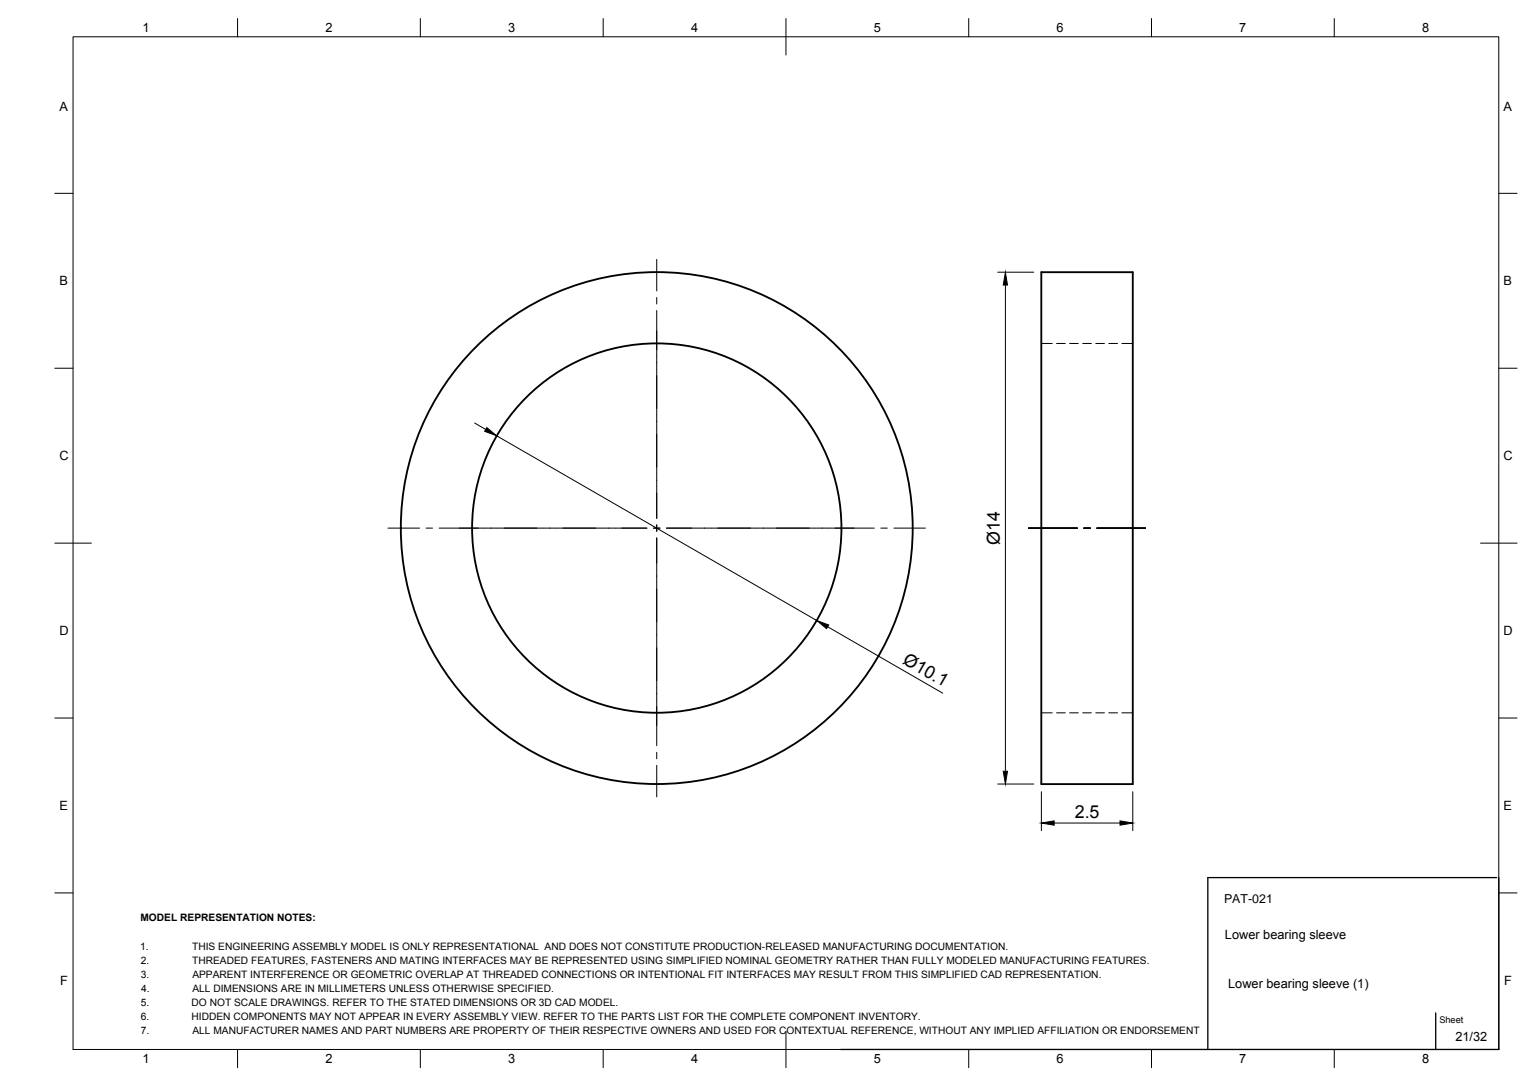
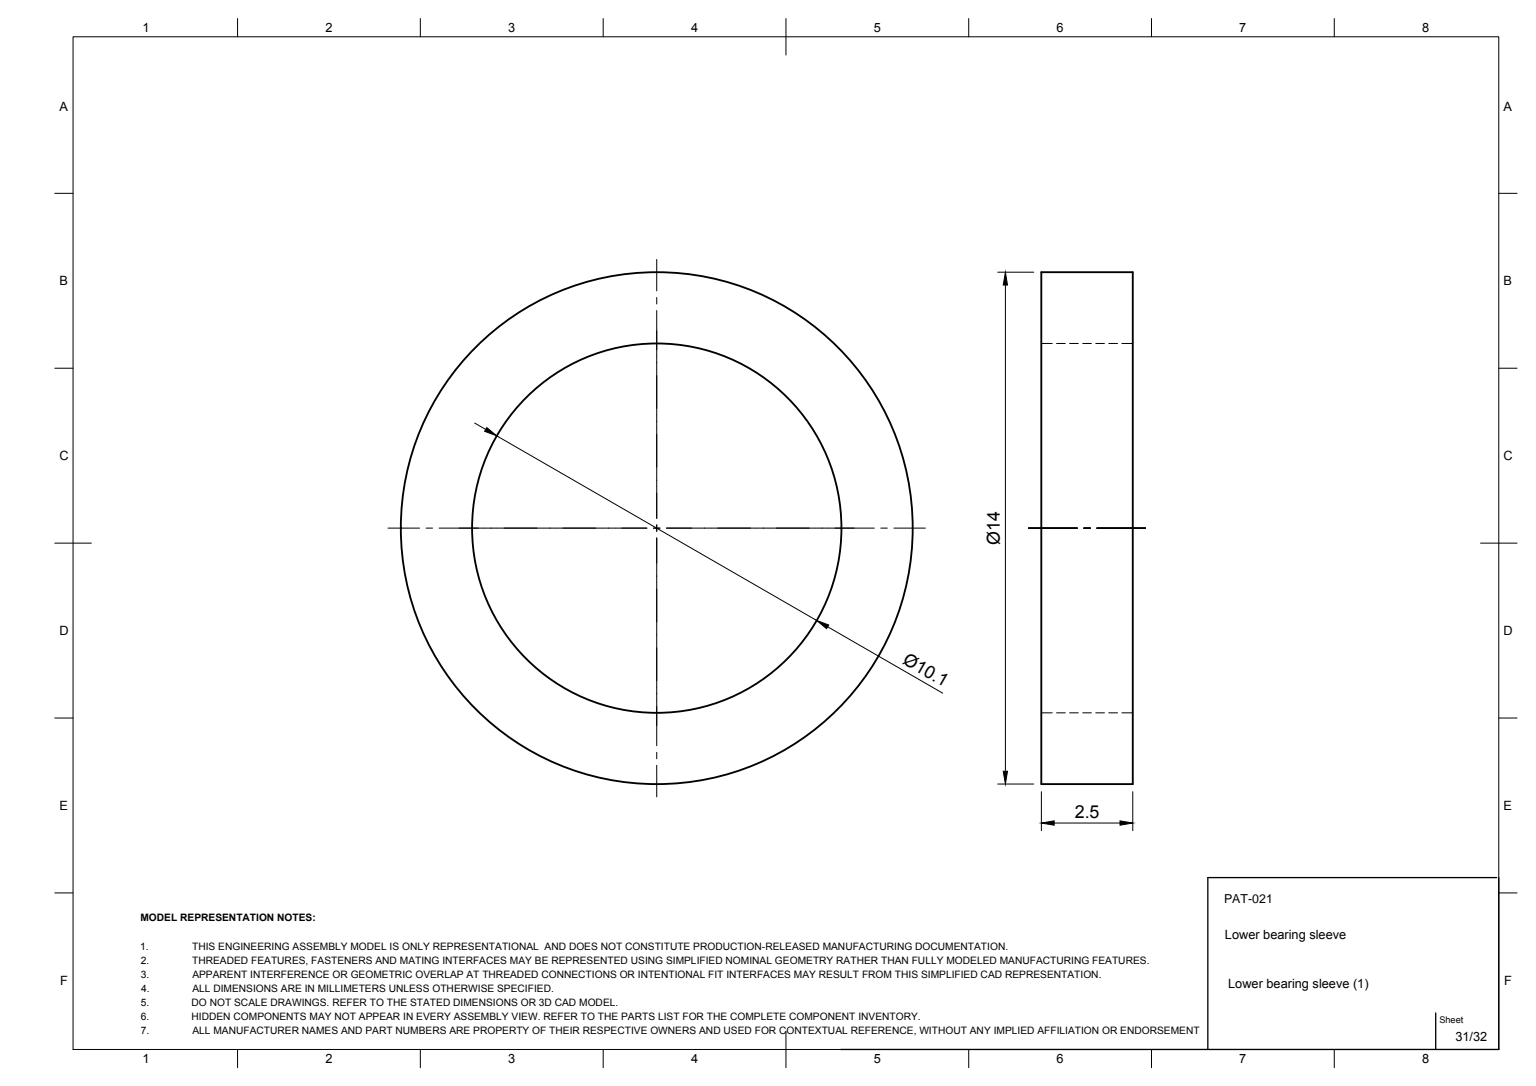
ISO-10303-21;
HEADER;
/* Generated by software containing ST-Developer
 * from STEP Tools, Inc. (www.steptools.com) 
 */

FILE_DESCRIPTION(
/* description */ ('Chain-less indexing wheel (Geneva) drive'),
/* implementation_level */ '2;1');

FILE_NAME(
/* name */ 'Lower bearing sleeve.step',
/* time_stamp */ '2026-10-28T03:25:22-07:00',
/* author */ (''),
/* organization */ (''),
/* preprocessor_version */ 'ST-DEVELOPER v20.2',
/* originating_system */ 'Autodesk Translation Framework v15.17.0.0',
/* authorisation */ '');

FILE_SCHEMA (('AUTOMOTIVE_DESIGN { 1 0 10303 214 3 1 1 }'));
ENDSEC;

DATA;
#10=MECHANICAL_DESIGN_GEOMETRIC_PRESENTATION_REPRESENTATION('',(#324),#10957);
#266=SHAPE_REPRESENTATION_RELATIONSHIP('SRR','None',#11081,#291);
#291=ADVANCED_BREP_SHAPE_REPRESENTATION('',(#356),#10944);
#324=STYLED_ITEM('',(#11287),#356);
#356=MANIFOLD_SOLID_BREP('Body1',#5721);
#439=FACE_BOUND('',#1255,.T.);
#440=FACE_BOUND('',#1257,.T.);
#567=PLANE('',#6448);
#568=PLANE('',#6449);
#847=FACE_OUTER_BOUND('',#1252,.T.);
#848=FACE_OUTER_BOUND('',#1253,.T.);
#849=FACE_OUTER_BOUND('',#1254,.T.);
#850=FACE_OUTER_BOUND('',#1256,.T.);
#1252=EDGE_LOOP('',(#4589,#4590,#4591,#4592));
#1253=EDGE_LOOP('',(#4593,#4594,#4595,#4596));
#1254=EDGE_LOOP('',(#4597));
#1255=EDGE_LOOP('',(#4598));
#1256=EDGE_LOOP('',(#4599));
#1257=EDGE_LOOP('',(#4600));
#1610=LINE('',#9926,#1984);
#1611=LINE('',#9932,#1985);
#1984=VECTOR('',#7804,0.505);
#1985=VECTOR('',#7811,0.7);
#2385=CIRCLE('',#6443,0.505);
#2386=CIRCLE('',#6444,0.505);
#2387=CIRCLE('',#6446,0.7);
#2388=CIRCLE('',#6447,0.7);
#2783=VERTEX_POINT('',#9923);
#2784=VERTEX_POINT('',#9925);
#2785=VERTEX_POINT('',#9929);
#2786=VERTEX_POINT('',#9931);
#3420=EDGE_CURVE('',#2783,#2783,#2385,.T.);
#3421=EDGE_CURVE('',#2783,#2784,#1610,.T.);
#3422=EDGE_CURVE('',#2784,#2784,#2386,.T.);
#3423=EDGE_CURVE('',#2785,#2785,#2387,.T.);
#3424=EDGE_CURVE('',#2785,#2786,#1611,.T.);
#3425=EDGE_CURVE('',#2786,#2786,#2388,.T.);
#4589=ORIENTED_EDGE('',*,*,#3420,.F.);
#4590=ORIENTED_EDGE('',*,*,#3421,.T.);
#4591=ORIENTED_EDGE('',*,*,#3422,.T.);
#4592=ORIENTED_EDGE('',*,*,#3421,.F.);
#4593=ORIENTED_EDGE('',*,*,#3423,.F.);
#4594=ORIENTED_EDGE('',*,*,#3424,.T.);
#4595=ORIENTED_EDGE('',*,*,#3425,.T.);
#4596=ORIENTED_EDGE('',*,*,#3424,.F.);
#4597=ORIENTED_EDGE('',*,*,#3423,.T.);
#4598=ORIENTED_EDGE('',*,*,#3420,.T.);
#4599=ORIENTED_EDGE('',*,*,#3425,.F.);
#4600=ORIENTED_EDGE('',*,*,#3422,.F.);
#5317=CYLINDRICAL_SURFACE('',#6442,0.505);
#5318=CYLINDRICAL_SURFACE('',#6445,0.7);
#5561=ADVANCED_FACE('',(#847),#5317,.F.);
#5562=ADVANCED_FACE('',(#848),#5318,.T.);
#5563=ADVANCED_FACE('',(#849,#439),#567,.T.);
#5564=ADVANCED_FACE('',(#850,#440),#568,.F.);
#5721=CLOSED_SHELL('',(#5561,#5562,#5563,#5564));
#6441=AXIS2_PLACEMENT_3D('',#9921,#7798,#7799);
#6442=AXIS2_PLACEMENT_3D('',#9922,#7800,#7801);
#6443=AXIS2_PLACEMENT_3D('',#9924,#7802,#7803);
#6444=AXIS2_PLACEMENT_3D('',#9927,#7805,#7806);
#6445=AXIS2_PLACEMENT_3D('',#9928,#7807,#7808);
#6446=AXIS2_PLACEMENT_3D('',#9930,#7809,#7810);
#6447=AXIS2_PLACEMENT_3D('',#9933,#7812,#7813);
#6448=AXIS2_PLACEMENT_3D('',#9934,#7814,#7815);
#6449=AXIS2_PLACEMENT_3D('',#9935,#7816,#7817);
#7798=DIRECTION('axis',(0.,0.,1.));
#7799=DIRECTION('refdir',(1.,0.,0.));
#7800=DIRECTION('center_axis',(0.,0.,1.));
#7801=DIRECTION('ref_axis',(1.,0.,0.));
#7802=DIRECTION('center_axis',(0.,0.,-1.));
#7803=DIRECTION('ref_axis',(1.,0.,0.));
#7804=DIRECTION('',(0.,0.,-1.));
#7805=DIRECTION('center_axis',(0.,0.,-1.));
#7806=DIRECTION('ref_axis',(1.,0.,0.));
#7807=DIRECTION('center_axis',(0.,0.,1.));
#7808=DIRECTION('ref_axis',(1.,0.,0.));
#7809=DIRECTION('center_axis',(0.,0.,1.));
#7810=DIRECTION('ref_axis',(1.,0.,0.));
#7811=DIRECTION('',(0.,0.,-1.));
#7812=DIRECTION('center_axis',(0.,0.,1.));
#7813=DIRECTION('ref_axis',(1.,0.,0.));
#7814=DIRECTION('center_axis',(0.,0.,1.));
#7815=DIRECTION('ref_axis',(1.,0.,0.));
#7816=DIRECTION('center_axis',(0.,0.,1.));
#7817=DIRECTION('ref_axis',(1.,0.,0.));
#9921=CARTESIAN_POINT('',(0.,0.,0.));
#9922=CARTESIAN_POINT('Origin',(0.,0.,1.8));
#9923=CARTESIAN_POINT('',(-0.505,-6.18446633569413E-17,2.05));
#9924=CARTESIAN_POINT('Origin',(0.,0.,2.05));
#9925=CARTESIAN_POINT('',(-0.505,-6.18446633569413E-17,1.8));
#9926=CARTESIAN_POINT('',(-0.505,-6.18446633569413E-17,1.8));
#9927=CARTESIAN_POINT('Origin',(0.,0.,1.8));
#9928=CARTESIAN_POINT('Origin',(0.,0.,1.8));
#9929=CARTESIAN_POINT('',(-0.7,-8.57252759403147E-17,2.05));
#9930=CARTESIAN_POINT('Origin',(0.,0.,2.05));
#9931=CARTESIAN_POINT('',(-0.7,-8.57252759403147E-17,1.8));
#9932=CARTESIAN_POINT('',(-0.7,-8.57252759403147E-17,1.8));
#9933=CARTESIAN_POINT('Origin',(0.,0.,1.8));
#9934=CARTESIAN_POINT('Origin',(0.,0.,2.05));
#9935=CARTESIAN_POINT('Origin',(0.,0.,1.8));
#10913=UNCERTAINTY_MEASURE_WITH_UNIT(LENGTH_MEASURE(0.001),#10958,
'DISTANCE_ACCURACY_VALUE',
'Maximum model space distance between geometric entities at asserted c
onnectivities');
#10926=UNCERTAINTY_MEASURE_WITH_UNIT(LENGTH_MEASURE(0.001),#10958,
'DISTANCE_ACCURACY_VALUE',
'Maximum model space distance between geometric entities at asserted c
onnectivities');
#10944=(
GEOMETRIC_REPRESENTATION_CONTEXT(3)
GLOBAL_UNCERTAINTY_ASSIGNED_CONTEXT((#10913))
GLOBAL_UNIT_ASSIGNED_CONTEXT((#10958,#10960,#10961))
REPRESENTATION_CONTEXT('','3D')
);
#10957=(
GEOMETRIC_REPRESENTATION_CONTEXT(3)
GLOBAL_UNCERTAINTY_ASSIGNED_CONTEXT((#10926))
GLOBAL_UNIT_ASSIGNED_CONTEXT((#10958,#10960,#10961))
REPRESENTATION_CONTEXT('','3D')
);
#10958=(
LENGTH_UNIT()
NAMED_UNIT(*)
SI_UNIT(.CENTI.,.METRE.)
);
#10960=(
NAMED_UNIT(*)
PLANE_ANGLE_UNIT()
SI_UNIT($,.RADIAN.)
);
#10961=(
NAMED_UNIT(*)
SI_UNIT($,.STERADIAN.)
SOLID_ANGLE_UNIT()
);
#10979=SHAPE_DEFINITION_REPRESENTATION(#11014,#11081);
#11014=PRODUCT_DEFINITION_SHAPE('',$,#11112);
#11081=SHAPE_REPRESENTATION('',(#6441),#10944);
#11094=PRODUCT_DEFINITION_CONTEXT('part definition',#11186,'design');
#11112=PRODUCT_DEFINITION('Lower bearing sleeve','Lower bearing sleeve',
#11142,#11094);
#11142=PRODUCT_DEFINITION_FORMATION('',$,#11205);
#11186=APPLICATION_CONTEXT(
'Core Data for Automotive Mechanical Design Process');
#11187=PRODUCT_CONTEXT('part definition',#11186,'mechanical');
#11205=PRODUCT('Lower bearing sleeve','Lower bearing sleeve',
'Lower bearing sleeve',(#11187));
#11281=COLOUR_RGB('Grey',0.48,0.52,0.57);
#11282=FILL_AREA_STYLE_COLOUR('',#11281);
#11283=FILL_AREA_STYLE('',(#11282));
#11284=SURFACE_STYLE_FILL_AREA(#11283);
#11285=SURFACE_SIDE_STYLE('',(#11284));
#11286=SURFACE_STYLE_USAGE(.BOTH.,#11285);
#11287=PRESENTATION_STYLE_ASSIGNMENT((#11286));
ENDSEC;
END-ISO-10303-21;
